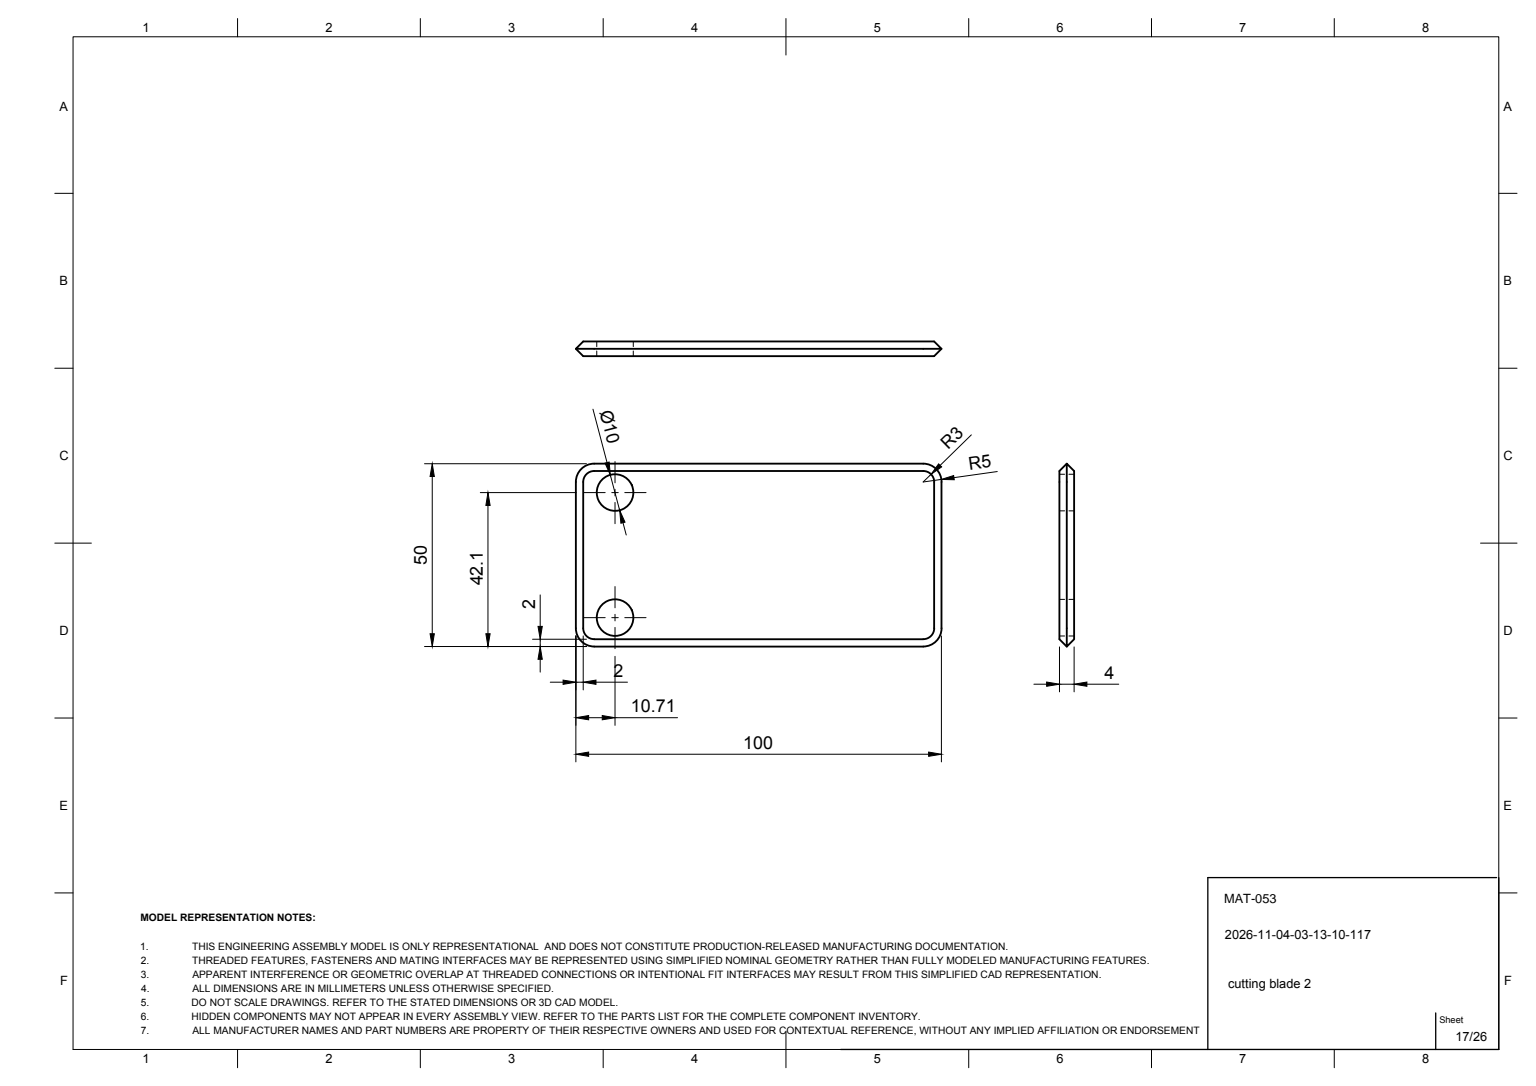
ISO-10303-21;
HEADER;
FILE_DESCRIPTION (('STEP AP214'),
    '1' );
FILE_NAME ('cutting blade 2.step',
    '2026-10-10T03:43:58',
    ( '' ),
    ( '' ),
    'SwSTEP 2.0',
    'SolidWorks 2026',
    '' );
FILE_SCHEMA (( 'AUTOMOTIVE_DESIGN' ));
ENDSEC;

DATA;
#183=ORIENTED_EDGE ( 'NONE', *, *, #3422, .F. ) ;
#222=LINE ( 'NONE', #22031, #68846 ) ;
#377=FACE_OUTER_BOUND ( 'NONE', #67584, .T. ) ;
#390=DIRECTION ( 'NONE',  ( 1.000000000000000000, 0.000000000000000000, 0.000000000000000000 ) ) ;
#471=LINE ( 'NONE', #21919, #18113 ) ;
#708=CARTESIAN_POINT ( 'NONE',  ( -48.00000000000000000, 19.99999999999996447, 0.000000000000000000 ) ) ;
#750=CARTESIAN_POINT ( 'NONE',  ( 44.99999999999997158, 22.99999999999998579, 0.000000000000000000 ) ) ;
#923=DIRECTION ( 'NONE',  ( -0.7071067811865463515, 0.000000000000000000, -0.7071067811865487940 ) ) ;
#986=EDGE_CURVE ( 'NONE', #12560, #40674, #59640, .T. ) ;
#1018=ORIENTED_EDGE ( 'NONE', *, *, #5991, .T. ) ;
#1098=DIRECTION ( 'NONE',  ( -4.906538933386759377E-15, 0.7071067811865474617, 0.7071067811865474617 ) ) ;
#1150=EDGE_LOOP ( 'NONE', ( #20877, #65074, #12430, #64337 ) ) ;
#1202=DIRECTION ( 'NONE',  ( 0.000000000000000000, 1.000000000000000000, -0.000000000000000000 ) ) ;
#1336=DIRECTION ( 'NONE',  ( 1.000000000000000000, 0.000000000000000000, 0.000000000000000000 ) ) ;
#1358=CARTESIAN_POINT ( 'NONE',  ( 49.99999999999998579, -19.99999999999996447, 2.000000000000015543 ) ) ;
#1404=DIRECTION ( 'NONE',  ( -0.000000000000000000, -0.000000000000000000, 1.000000000000000000 ) ) ;
#1589=CIRCLE ( 'NONE', #19567, 4.999999999999997335 ) ;
#1634=VECTOR ( 'NONE', #40606, 1000.000000000000114 ) ;
#1690=ORIENTED_EDGE ( 'NONE', *, *, #44656, .F. ) ;
#1791=AXIS2_PLACEMENT_3D ( 'NONE', #65034, #34080, #59734 ) ;
#2120=VERTEX_POINT ( 'NONE', #13833 ) ;
#2139=CARTESIAN_POINT ( 'NONE',  ( -44.29440389294402536, -17.09499999999999886, 0.000000000000000000 ) ) ;
#2256=EDGE_LOOP ( 'NONE', ( #42855, #11599, #67261, #3883 ) ) ;
#2297=CARTESIAN_POINT ( 'NONE',  ( 44.99999999999995737, -25.00000000000000000, 1.999999999999984457 ) ) ;
#2427=ORIENTED_EDGE ( 'NONE', *, *, #48014, .T. ) ;
#2635=CARTESIAN_POINT ( 'NONE',  ( -34.29440389294403246, 17.09499999999999886, 0.000000000000000000 ) ) ;
#2643=AXIS2_PLACEMENT_3D ( 'NONE', #60950, #23670, #66257 ) ;
#2797=CARTESIAN_POINT ( 'NONE',  ( -50.00000000000001421, -20.00000000000000355, 2.000000000000015543 ) ) ;
#2853=DIRECTION ( 'NONE',  ( -0.000000000000000000, -0.000000000000000000, -1.000000000000000000 ) ) ;
#2867=EDGE_LOOP ( 'NONE', ( #46115, #49842, #4255, #13345, #54855, #50718, #48598, #4064 ) ) ;
#2964=DIRECTION ( 'NONE',  ( -0.000000000000000000, -0.000000000000000000, -1.000000000000000000 ) ) ;
#3009=CARTESIAN_POINT ( 'NONE',  ( 44.99999999999995737, 25.00000000000000000, 1.999999999999984457 ) ) ;
#3125=CARTESIAN_POINT ( 'NONE',  ( 44.99999999999999289, -20.00000000000000355, 0.000000000000000000 ) ) ;
#3311=AXIS2_PLACEMENT_3D ( 'NONE', #56545, #46328, #29819 ) ;
#3422=EDGE_CURVE ( 'NONE', #60851, #22871, #1589, .T. ) ;
#3529=DIRECTION ( 'NONE',  ( -0.7071067811865474617, -4.906538933386759377E-15, 0.7071067811865474617 ) ) ;
#3745=AXIS2_PLACEMENT_3D ( 'NONE', #53453, #68615, #21797 ) ;
#3883=ORIENTED_EDGE ( 'NONE', *, *, #65380, .F. ) ;
#4036=EDGE_CURVE ( 'NONE', #50267, #15307, #38531, .T. ) ;
#4064=ORIENTED_EDGE ( 'NONE', *, *, #62499, .T. ) ;
#4223=CIRCLE ( 'NONE', #47977, 4.999999999999997335 ) ;
#4244=VERTEX_POINT ( 'NONE', #15155 ) ;
#4255=ORIENTED_EDGE ( 'NONE', *, *, #21903, .T. ) ;
#4322=ADVANCED_FACE ( 'NONE', ( #27075 ), #64387, .T. ) ;
#4732=CIRCLE ( 'NONE', #44038, 4.999999999999997335 ) ;
#4762=ORIENTED_EDGE ( 'NONE', *, *, #33113, .F. ) ;
#4799=VECTOR ( 'NONE', #923, 1000.000000000000000 ) ;
#4847=ADVANCED_FACE ( 'NONE', ( #5297 ), #68957, .T. ) ;
#4868=ADVANCED_FACE ( 'NONE', ( #22170 ), #20779, .T. ) ;
#4880=CARTESIAN_POINT ( 'NONE',  ( -39.29440389294403246, -17.09499999999999886, 4.000000000000000000 ) ) ;
#4934=CARTESIAN_POINT ( 'NONE',  ( -44.99999999999998579, 25.00000000000000000, 1.999999999999984457 ) ) ;
#4944=VERTEX_POINT ( 'NONE', #59784 ) ;
#5118=VECTOR ( 'NONE', #13219, 1000.000000000000114 ) ;
#5158=EDGE_CURVE ( 'NONE', #15307, #27145, #61873, .T. ) ;
#5229=DIRECTION ( 'NONE',  ( 0.000000000000000000, 0.000000000000000000, 1.000000000000000000 ) ) ;
#5297=FACE_OUTER_BOUND ( 'NONE', #5578, .T. ) ;
#5578=EDGE_LOOP ( 'NONE', ( #1690, #69065, #8868, #53921 ) ) ;
#5608=CARTESIAN_POINT ( 'NONE',  ( -45.00000000000002132, -20.00000000000000355, 2.000000000000015543 ) ) ;
#5732=CIRCLE ( 'NONE', #61882, 4.999999999999997335 ) ;
#5991=EDGE_CURVE ( 'NONE', #38832, #12486, #8955, .T. ) ;
#6249=EDGE_LOOP ( 'NONE', ( #30382, #9819, #17773, #59788 ) ) ;
#6275=DIRECTION ( 'NONE',  ( 0.000000000000000000, -1.000000000000000000, 0.000000000000000000 ) ) ;
#6382=CARTESIAN_POINT ( 'NONE',  ( -50.00000000000001421, 19.99999999999996447, 1.999999999999984457 ) ) ;
#6523=DIRECTION ( 'NONE',  ( -1.000000000000000000, 0.000000000000000000, 0.000000000000000000 ) ) ;
#6705=DIRECTION ( 'NONE',  ( -0.000000000000000000, -0.000000000000000000, -1.000000000000000000 ) ) ;
#6931=PRODUCT_CONTEXT ( 'NONE', #28708, 'mechanical' ) ;
#6943=DIRECTION ( 'NONE',  ( -1.000000000000000000, 0.000000000000000000, 0.000000000000000000 ) ) ;
#7122=CARTESIAN_POINT ( 'NONE',  ( 44.99999999999995737, -25.00000000000000000, 1.999999999999984457 ) ) ;
#7235=EDGE_CURVE ( 'NONE', #28864, #10266, #16985, .T. ) ;
#7533=DIRECTION ( 'NONE',  ( -0.000000000000000000, 0.7071067811865475727, 0.7071067811865475727 ) ) ;
#7537=VERTEX_POINT ( 'NONE', #53319 ) ;
#7773=DIRECTION ( 'NONE',  ( -0.000000000000000000, -0.000000000000000000, 1.000000000000000000 ) ) ;
#7845=CARTESIAN_POINT ( 'NONE',  ( -45.00000000000002132, 20.00000000000000355, 2.000000000000015543 ) ) ;
#7877=LINE ( 'NONE', #61339, #37506 ) ;
#7900=DIRECTION ( 'NONE',  ( 1.000000000000000000, 0.000000000000000000, 0.000000000000000000 ) ) ;
#8025=CARTESIAN_POINT ( 'NONE',  ( -34.29440389294403246, 17.09499999999999886, 4.000000000000000000 ) ) ;
#8072=CARTESIAN_POINT ( 'NONE',  ( -34.29440389294403246, -17.09499999999999886, 4.000000000000000000 ) ) ;
#8319=DIRECTION ( 'NONE',  ( 1.000000000000000000, 0.000000000000000000, 0.000000000000000000 ) ) ;
#8398=FACE_BOUND ( 'NONE', #48504, .T. ) ;
#8425=EDGE_CURVE ( 'NONE', #35305, #28864, #65814, .T. ) ;
#8459=AXIS2_PLACEMENT_3D ( 'NONE', #30320, #9554, #52459 ) ;
#8475=SURFACE_STYLE_FILL_AREA ( #51035 ) ;
#8515=VECTOR ( 'NONE', #8859, 1000.000000000000114 ) ;
#8610=CYLINDRICAL_SURFACE ( 'NONE', #31391, 4.999999999999997335 ) ;
#8770=( NAMED_UNIT ( * ) SI_UNIT ( $, .STERADIAN. ) SOLID_ANGLE_UNIT ( ) );
#8823=ORIENTED_EDGE ( 'NONE', *, *, #5158, .T. ) ;
#8843=CARTESIAN_POINT ( 'NONE',  ( -34.29440389294403246, -17.09499999999999886, 4.000000000000000000 ) ) ;
#8859=DIRECTION ( 'NONE',  ( 0.7071067811865474617, 0.000000000000000000, -0.7071067811865474617 ) ) ;
#8868=ORIENTED_EDGE ( 'NONE', *, *, #31433, .F. ) ;
#8955=LINE ( 'NONE', #2297, #1634 ) ;
#9255=ORIENTED_EDGE ( 'NONE', *, *, #36424, .T. ) ;
#9426=AXIS2_PLACEMENT_3D ( 'NONE', #64039, #26413, #64375 ) ;
#9467=CONICAL_SURFACE ( 'NONE', #13979, 4.999999999999997335, 0.7853981633974482790 ) ;
#9554=DIRECTION ( 'NONE',  ( 0.000000000000000000, 0.000000000000000000, -1.000000000000000000 ) ) ;
#9615=VECTOR ( 'NONE', #7900, 1000.000000000000000 ) ;
#9738=LINE ( 'NONE', #67202, #34763 ) ;
#9744=ORIENTED_EDGE ( 'NONE', *, *, #46447, .T. ) ;
#9800=ORIENTED_EDGE ( 'NONE', *, *, #50666, .T. ) ;
#9819=ORIENTED_EDGE ( 'NONE', *, *, #48014, .F. ) ;
#10092=CARTESIAN_POINT ( 'NONE',  ( 47.99999999999997158, 19.99999999999996447, 4.000000000000000000 ) ) ;
#10095=CIRCLE ( 'NONE', #43771, 4.999999999999997335 ) ;
#10266=VERTEX_POINT ( 'NONE', #11721 ) ;
#10705=PLANE ( 'NONE',  #20640 ) ;
#11124=DIRECTION ( 'NONE',  ( -0.7071067811865474617, 0.000000000000000000, 0.7071067811865474617 ) ) ;
#11164=CARTESIAN_POINT ( 'NONE',  ( 47.99999999999997158, 19.99999999999996447, 4.000000000000000000 ) ) ;
#11274=CARTESIAN_POINT ( 'NONE',  ( -34.29440389294403246, 17.09499999999999886, 4.000000000000000000 ) ) ;
#11390=CARTESIAN_POINT ( 'NONE',  ( 49.99999999999998579, -19.99999999999996447, 2.000000000000015543 ) ) ;
#11409=DIRECTION ( 'NONE',  ( 0.000000000000000000, 1.000000000000000000, 0.000000000000000000 ) ) ;
#11454=CARTESIAN_POINT ( 'NONE',  ( -48.00000000000000711, -20.00000000000000355, 4.000000000000000000 ) ) ;
#11599=ORIENTED_EDGE ( 'NONE', *, *, #4036, .F. ) ;
#11721=CARTESIAN_POINT ( 'NONE',  ( -44.29440389294402536, 17.09499999999999886, 0.000000000000000000 ) ) ;
#11786=FACE_OUTER_BOUND ( 'NONE', #1150, .T. ) ;
#11882=DIRECTION ( 'NONE',  ( 0.000000000000000000, 0.000000000000000000, 1.000000000000000000 ) ) ;
#12224=CARTESIAN_POINT ( 'NONE',  ( 44.99999999999999289, 20.00000000000000355, 4.000000000000000000 ) ) ;
#12325=VECTOR ( 'NONE', #37666, 1000.000000000000000 ) ;
#12430=ORIENTED_EDGE ( 'NONE', *, *, #5991, .F. ) ;
#12479=DIRECTION ( 'NONE',  ( 4.906538933386759377E-15, 0.7071067811865474617, -0.7071067811865474617 ) ) ;
#12486=VERTEX_POINT ( 'NONE', #28146 ) ;
#12522=VECTOR ( 'NONE', #11409, 1000.000000000000000 ) ;
#12560=VERTEX_POINT ( 'NONE', #44325 ) ;
#12589=ORIENTED_EDGE ( 'NONE', *, *, #62499, .F. ) ;
#12741=DIRECTION ( 'NONE',  ( 0.000000000000000000, 0.000000000000000000, 1.000000000000000000 ) ) ;
#12788=EDGE_CURVE ( 'NONE', #35305, #62075, #59114, .T. ) ;
#12803=CARTESIAN_POINT ( 'NONE',  ( -44.99999999999998579, -25.00000000000000000, 2.000000000000015543 ) ) ;
#12850=DIRECTION ( 'NONE',  ( -0.000000000000000000, -0.000000000000000000, -1.000000000000000000 ) ) ;
#12851=VERTEX_POINT ( 'NONE', #22536 ) ;
#12994=CARTESIAN_POINT ( 'NONE',  ( -44.99999999999998579, 25.00000000000000000, 2.000000000000015543 ) ) ;
#13009=ORIENTED_EDGE ( 'NONE', *, *, #49203, .T. ) ;
#13019=FACE_OUTER_BOUND ( 'NONE', #6249, .T. ) ;
#13037=DIRECTION ( 'NONE',  ( -0.000000000000000000, -0.000000000000000000, 1.000000000000000000 ) ) ;
#13138=FACE_OUTER_BOUND ( 'NONE', #28425, .T. ) ;
#13214=EDGE_CURVE ( 'NONE', #16065, #15985, #21273, .T. ) ;
#13219=DIRECTION ( 'NONE',  ( 4.906538933386759377E-15, -0.7071067811865474617, 0.7071067811865474617 ) ) ;
#13345=ORIENTED_EDGE ( 'NONE', *, *, #48539, .T. ) ;
#13488=AXIS2_PLACEMENT_3D ( 'NONE', #22899, #7773, #17980 ) ;
#13502=EDGE_CURVE ( 'NONE', #63560, #2120, #43992, .T. ) ;
#13538=CARTESIAN_POINT ( 'NONE',  ( -44.99999999999998579, 25.00000000000000000, 2.000000000000015543 ) ) ;
#13780=CARTESIAN_POINT ( 'NONE',  ( 44.99999999999999289, -20.00000000000000355, 2.000000000000015543 ) ) ;
#13831=DIRECTION ( 'NONE',  ( 0.000000000000000000, 0.000000000000000000, 1.000000000000000000 ) ) ;
#13833=CARTESIAN_POINT ( 'NONE',  ( 44.99999999999995737, 25.00000000000000000, 1.999999999999984457 ) ) ;
#13881=EDGE_CURVE ( 'NONE', #4944, #25496, #66247, .T. ) ;
#13979=AXIS2_PLACEMENT_3D ( 'NONE', #5608, #47479, #52756 ) ;
#14090=LINE ( 'NONE', #52413, #14981 ) ;
#14258=PLANE ( 'NONE',  #28801 ) ;
#14352=DIRECTION ( 'NONE',  ( 0.000000000000000000, -0.7071067811865474617, -0.7071067811865474617 ) ) ;
#14380=AXIS2_PLACEMENT_3D ( 'NONE', #24758, #63424, #57113 ) ;
#14790=AXIS2_PLACEMENT_3D ( 'NONE', #30257, #24641, #63650 ) ;
#14981=VECTOR ( 'NONE', #3529, 1000.000000000000114 ) ;
#14989=ORIENTED_EDGE ( 'NONE', *, *, #7235, .T. ) ;
#14998=ADVANCED_FACE ( 'NONE', ( #61511, #8398, #60802 ), #50261, .F. ) ;
#15004=DIRECTION ( 'NONE',  ( 0.000000000000000000, -1.000000000000000000, 0.000000000000000000 ) ) ;
#15155=CARTESIAN_POINT ( 'NONE',  ( -44.99999999999998579, -25.00000000000000000, 1.999999999999984457 ) ) ;
#15307=VERTEX_POINT ( 'NONE', #60726 ) ;
#15476=SURFACE_STYLE_USAGE ( .BOTH. , #52740 ) ;
#15509=EDGE_LOOP ( 'NONE', ( #32307, #42326, #26888, #23575 ) ) ;
#15809=PRESENTATION_STYLE_ASSIGNMENT (( #15476 ) ) ;
#15831=AXIS2_PLACEMENT_3D ( 'NONE', #19106, #13831, #18417 ) ;
#15947=CLOSED_SHELL ( 'NONE', ( #32652, #33942, #58809, #14998, #32048, #67428, #50501, #38188, #4847, #4322, #43169, #65687, #64587, #40447, #23137, #4868, #26968, #20171, #36132, #26544, #66069, #55190 ) ) ;
#15985=VERTEX_POINT ( 'NONE', #68162 ) ;
#16065=VERTEX_POINT ( 'NONE', #10092 ) ;
#16112=EDGE_LOOP ( 'NONE', ( #27726, #56434 ) ) ;
#16253=PRODUCT_DEFINITION_CONTEXT ( 'detailed design', #53830, 'design' ) ;
#16512=ORIENTED_EDGE ( 'NONE', *, *, #32179, .T. ) ;
#16541=FACE_OUTER_BOUND ( 'NONE', #31950, .T. ) ;
#16985=LINE ( 'NONE', #49686, #46669 ) ;
#17050=CARTESIAN_POINT ( 'NONE',  ( 47.99999999999997158, -19.99999999999997868, 0.000000000000000000 ) ) ;
#17127=EDGE_CURVE ( 'NONE', #25708, #50267, #25270, .T. ) ;
#17166=COLOUR_RGB ( '',0.7921568627450980005, 0.8196078431372548767, 0.9333333333333333481 ) ;
#17773=ORIENTED_EDGE ( 'NONE', *, *, #25587, .F. ) ;
#17789=VECTOR ( 'NONE', #12479, 1000.000000000000114 ) ;
#17937=DIRECTION ( 'NONE',  ( -0.000000000000000000, -0.000000000000000000, -1.000000000000000000 ) ) ;
#17980=DIRECTION ( 'NONE',  ( 1.000000000000000000, 0.000000000000000000, 0.000000000000000000 ) ) ;
#18104=CARTESIAN_POINT ( 'NONE',  ( 44.99999999999995737, -22.99999999999998579, 4.000000000000000000 ) ) ;
#18113=VECTOR ( 'NONE', #44422, 1000.000000000000114 ) ;
#18224=DIRECTION ( 'NONE',  ( 0.000000000000000000, -1.000000000000000000, 0.000000000000000000 ) ) ;
#18228=ORIENTED_EDGE ( 'NONE', *, *, #51150, .F. ) ;
#18296=FACE_OUTER_BOUND ( 'NONE', #2256, .T. ) ;
#18356=EDGE_CURVE ( 'NONE', #40674, #18627, #20345, .T. ) ;
#18417=DIRECTION ( 'NONE',  ( 1.000000000000000000, 0.000000000000000000, 0.000000000000000000 ) ) ;
#18522=DIRECTION ( 'NONE',  ( -0.000000000000000000, -0.000000000000000000, 1.000000000000000000 ) ) ;
#18580=CARTESIAN_POINT ( 'NONE',  ( -45.00000000000002132, 20.00000000000000355, 4.000000000000000000 ) ) ;
#18627=VERTEX_POINT ( 'NONE', #41386 ) ;
#18718=DIRECTION ( 'NONE',  ( 1.000000000000000000, 0.000000000000000000, 0.000000000000000000 ) ) ;
#18762=ORIENTED_EDGE ( 'NONE', *, *, #23426, .F. ) ;
#18857=ORIENTED_EDGE ( 'NONE', *, *, #13881, .F. ) ;
#18879=SHAPE_DEFINITION_REPRESENTATION ( #51752, #64096 ) ;
#19106=CARTESIAN_POINT ( 'NONE',  ( -39.29440389294403246, -17.09499999999999886, 0.000000000000000000 ) ) ;
#19194=CIRCLE ( 'NONE', #59591, 4.999999999999997335 ) ;
#19282=DIRECTION ( 'NONE',  ( 0.000000000000000000, 0.000000000000000000, 1.000000000000000000 ) ) ;
#19376=CARTESIAN_POINT ( 'NONE',  ( -44.29440389294402536, 17.09499999999999886, 4.000000000000000000 ) ) ;
#19480=CARTESIAN_POINT ( 'NONE',  ( -45.00000000000000000, 22.99999999999998579, 4.000000000000000000 ) ) ;
#19491=CARTESIAN_POINT ( 'NONE',  ( -39.29440389294403246, -17.09499999999999886, 4.000000000000000000 ) ) ;
#19560=CARTESIAN_POINT ( 'NONE',  ( -44.99999999999998579, -25.00000000000000000, 2.000000000000015543 ) ) ;
#19567=AXIS2_PLACEMENT_3D ( 'NONE', #54925, #60906, #28914 ) ;
#19604=CARTESIAN_POINT ( 'NONE',  ( -50.00000000000001421, -19.99999999999996447, 2.000000000000015543 ) ) ;
#19746=LINE ( 'NONE', #57045, #8515 ) ;
#19766=LINE ( 'NONE', #56710, #40477 ) ;
#19850=PLANE ( 'NONE',  #63041 ) ;
#19933=EDGE_LOOP ( 'NONE', ( #24188, #34340, #56345, #65370 ) ) ;
#20171=ADVANCED_FACE ( 'NONE', ( #18296 ), #55242, .T. ) ;
#20217=DIRECTION ( 'NONE',  ( 0.000000000000000000, 0.000000000000000000, 1.000000000000000000 ) ) ;
#20278=EDGE_CURVE ( 'NONE', #22871, #60851, #4732, .T. ) ;
#20345=LINE ( 'NONE', #2797, #41653 ) ;
#20428=CARTESIAN_POINT ( 'NONE',  ( 47.99999999999997158, 19.99999999999996447, 0.000000000000000000 ) ) ;
#20585=CARTESIAN_POINT ( 'NONE',  ( 47.99999999999997158, 19.99999999999996447, 0.000000000000000000 ) ) ;
#20640=AXIS2_PLACEMENT_3D ( 'NONE', #11390, #49018, #1202 ) ;
#20779=PLANE ( 'NONE',  #28501 ) ;
#20844=VECTOR ( 'NONE', #62363, 1000.000000000000114 ) ;
#20877=ORIENTED_EDGE ( 'NONE', *, *, #67680, .T. ) ;
#20898=EDGE_LOOP ( 'NONE', ( #47431, #46905, #14989, #35358 ) ) ;
#20942=VECTOR ( 'NONE', #33017, 1000.000000000000000 ) ;
#21176=VERTEX_POINT ( 'NONE', #25603 ) ;
#21178=ORIENTED_EDGE ( 'NONE', *, *, #40498, .T. ) ;
#21271=EDGE_CURVE ( 'NONE', #42749, #16065, #222, .T. ) ;
#21273=CIRCLE ( 'NONE', #3311, 2.999999999999981792 ) ;
#21355=ORIENTED_EDGE ( 'NONE', *, *, #34936, .F. ) ;
#21466=DIRECTION ( 'NONE',  ( 0.000000000000000000, 1.000000000000000000, 0.000000000000000000 ) ) ;
#21508=ORIENTED_EDGE ( 'NONE', *, *, #36424, .F. ) ;
#21797=DIRECTION ( 'NONE',  ( 1.000000000000000000, 0.000000000000000000, 0.000000000000000000 ) ) ;
#21854=ORIENTED_EDGE ( 'NONE', *, *, #13502, .F. ) ;
#21903=EDGE_CURVE ( 'NONE', #12486, #21176, #62173, .T. ) ;
#21919=CARTESIAN_POINT ( 'NONE',  ( -44.99999999999998579, 25.00000000000000000, 2.000000000000015543 ) ) ;
#21973=LINE ( 'NONE', #65961, #12522 ) ;
#22005=AXIS2_PLACEMENT_3D ( 'NONE', #32747, #34156, #27111 ) ;
#22031=CARTESIAN_POINT ( 'NONE',  ( 49.99999999999998579, 19.99999999999996447, 1.999999999999984457 ) ) ;
#22079=DIRECTION ( 'NONE',  ( -0.000000000000000000, -0.000000000000000000, -1.000000000000000000 ) ) ;
#22170=FACE_OUTER_BOUND ( 'NONE', #63972, .T. ) ;
#22536=CARTESIAN_POINT ( 'NONE',  ( -45.00000000000000000, 22.99999999999998579, 0.000000000000000000 ) ) ;
#22658=UNCERTAINTY_MEASURE_WITH_UNIT (LENGTH_MEASURE( 1.000000000000000082E-05 ), #50619, 'distance_accuracy_value', 'NONE');
#22858=DIRECTION ( 'NONE',  ( 1.000000000000000000, 0.000000000000000000, 0.000000000000000000 ) ) ;
#22871=VERTEX_POINT ( 'NONE', #8843 ) ;
#22899=CARTESIAN_POINT ( 'NONE',  ( -45.00000000000002132, -20.00000000000000355, 2.000000000000015543 ) ) ;
#23124=VECTOR ( 'NONE', #51323, 1000.000000000000114 ) ;
#23130=DIRECTION ( 'NONE',  ( -0.000000000000000000, -0.000000000000000000, -1.000000000000000000 ) ) ;
#23137=ADVANCED_FACE ( 'NONE', ( #13138 ), #9467, .T. ) ;
#23379=EDGE_CURVE ( 'NONE', #25708, #42749, #68770, .T. ) ;
#23426=EDGE_CURVE ( 'NONE', #4244, #38832, #45946, .T. ) ;
#23485=CYLINDRICAL_SURFACE ( 'NONE', #45903, 4.999999999999997335 ) ;
#23575=ORIENTED_EDGE ( 'NONE', *, *, #27011, .F. ) ;
#23602=FACE_OUTER_BOUND ( 'NONE', #50503, .T. ) ;
#23670=DIRECTION ( 'NONE',  ( -0.000000000000000000, -0.000000000000000000, -1.000000000000000000 ) ) ;
#23733=ORIENTED_EDGE ( 'NONE', *, *, #20278, .T. ) ;
#23738=VECTOR ( 'NONE', #31568, 1000.000000000000000 ) ;
#23823=FACE_OUTER_BOUND ( 'NONE', #62051, .T. ) ;
#23895=SHAPE_REPRESENTATION_RELATIONSHIP ( 'NONE' , 'NONE' ,  #64096, #40723 ) ;
#24022=DIRECTION ( 'NONE',  ( 1.000000000000000000, 0.000000000000000000, 0.000000000000000000 ) ) ;
#24188=ORIENTED_EDGE ( 'NONE', *, *, #3422, .T. ) ;
#24480=ORIENTED_EDGE ( 'NONE', *, *, #48539, .F. ) ;
#24585=DIRECTION ( 'NONE',  ( 1.000000000000000000, 0.000000000000000000, -0.000000000000000000 ) ) ;
#24641=DIRECTION ( 'NONE',  ( -0.000000000000000000, -0.000000000000000000, -1.000000000000000000 ) ) ;
#24758=CARTESIAN_POINT ( 'NONE',  ( -45.00000000000002132, 20.00000000000000355, 0.000000000000000000 ) ) ;
#25032=EDGE_CURVE ( 'NONE', #65565, #12486, #60661, .T. ) ;
#25166=DIRECTION ( 'NONE',  ( 0.000000000000000000, 0.000000000000000000, 1.000000000000000000 ) ) ;
#25270=LINE ( 'NONE', #30198, #23738 ) ;
#25396=DIRECTION ( 'NONE',  ( 0.000000000000000000, 0.000000000000000000, -1.000000000000000000 ) ) ;
#25496=VERTEX_POINT ( 'NONE', #65880 ) ;
#25587=EDGE_CURVE ( 'NONE', #39558, #31561, #19746, .T. ) ;
#25603=CARTESIAN_POINT ( 'NONE',  ( 47.99999999999997158, -19.99999999999997868, 4.000000000000000000 ) ) ;
#25633=CIRCLE ( 'NONE', #14380, 2.999999999999981792 ) ;
#25708=VERTEX_POINT ( 'NONE', #20428 ) ;
#25725=CIRCLE ( 'NONE', #58246, 2.999999999999981792 ) ;
#26176=MECHANICAL_DESIGN_GEOMETRIC_PRESENTATION_REPRESENTATION('',(#58740),#28427);
#26257=CARTESIAN_POINT ( 'NONE',  ( -48.00000000000000711, -20.00000000000000355, 4.000000000000000000 ) ) ;
#26413=DIRECTION ( 'NONE',  ( 0.000000000000000000, 0.7071067811865475727, 0.7071067811865475727 ) ) ;
#26495=ORIENTED_EDGE ( 'NONE', *, *, #4036, .T. ) ;
#26544=ADVANCED_FACE ( 'NONE', ( #62322 ), #50018, .T. ) ;
#26865=AXIS2_PLACEMENT_3D ( 'NONE', #12224, #49484, #66749 ) ;
#26888=ORIENTED_EDGE ( 'NONE', *, *, #18356, .F. ) ;
#26968=ADVANCED_FACE ( 'NONE', ( #23602 ), #40806, .T. ) ;
#27011=EDGE_CURVE ( 'NONE', #39558, #40674, #54448, .T. ) ;
#27075=FACE_OUTER_BOUND ( 'NONE', #67313, .T. ) ;
#27085=DIRECTION ( 'NONE',  ( 0.000000000000000000, -0.7071067811865475727, 0.7071067811865475727 ) ) ;
#27111=DIRECTION ( 'NONE',  ( 1.000000000000000000, 0.000000000000000000, 0.000000000000000000 ) ) ;
#27145=VERTEX_POINT ( 'NONE', #62091 ) ;
#27228=FACE_OUTER_BOUND ( 'NONE', #54661, .T. ) ;
#27273=AXIS2_PLACEMENT_3D ( 'NONE', #30730, #2964, #46902 ) ;
#27455=EDGE_CURVE ( 'NONE', #25496, #39558, #40907, .T. ) ;
#27726=ORIENTED_EDGE ( 'NONE', *, *, #34770, .F. ) ;
#28146=CARTESIAN_POINT ( 'NONE',  ( 44.99999999999995737, -22.99999999999998579, 4.000000000000000000 ) ) ;
#28425=EDGE_LOOP ( 'NONE', ( #35121, #67993, #48370, #21355 ) ) ;
#28427=( GEOMETRIC_REPRESENTATION_CONTEXT ( 3 ) GLOBAL_UNCERTAINTY_ASSIGNED_CONTEXT ( ( #33920 ) ) GLOBAL_UNIT_ASSIGNED_CONTEXT ( ( #53424, #30620, #41516 ) ) REPRESENTATION_CONTEXT ( 'NONE', 'WORKASPACE' ) );
#28433=LINE ( 'NONE', #1358, #20942 ) ;
#28501=AXIS2_PLACEMENT_3D ( 'NONE', #36626, #42242, #21466 ) ;
#28708=APPLICATION_CONTEXT ( 'automotive_design' ) ;
#28801=AXIS2_PLACEMENT_3D ( 'NONE', #35717, #25166, #46595 ) ;
#28844=LINE ( 'NONE', #8072, #51936 ) ;
#28864=VERTEX_POINT ( 'NONE', #19376 ) ;
#28914=DIRECTION ( 'NONE',  ( 1.000000000000000000, 0.000000000000000000, 0.000000000000000000 ) ) ;
#28943=ORIENTED_EDGE ( 'NONE', *, *, #5158, .F. ) ;
#29154=AXIS2_PLACEMENT_3D ( 'NONE', #32742, #59461, #42932 ) ;
#29202=DIRECTION ( 'NONE',  ( 0.7071067811865474617, 4.906538933386759377E-15, 0.7071067811865474617 ) ) ;
#29271=ORIENTED_EDGE ( 'NONE', *, *, #45883, .F. ) ;
#29421=ORIENTED_EDGE ( 'NONE', *, *, #67680, .F. ) ;
#29435=ORIENTED_EDGE ( 'NONE', *, *, #45883, .T. ) ;
#29570=FILL_AREA_STYLE_COLOUR ( '', #17166 ) ;
#29663=DIRECTION ( 'NONE',  ( 1.000000000000000000, 0.000000000000000000, 0.000000000000000000 ) ) ;
#29819=DIRECTION ( 'NONE',  ( 1.000000000000000000, 0.000000000000000000, 0.000000000000000000 ) ) ;
#30184=CARTESIAN_POINT ( 'NONE',  ( -44.99999999999998579, -22.99999999999998579, 4.000000000000000000 ) ) ;
#30193=ORIENTED_EDGE ( 'NONE', *, *, #43361, .F. ) ;
#30198=CARTESIAN_POINT ( 'NONE',  ( 47.99999999999997158, -20.00000000000000355, 0.000000000000000000 ) ) ;
#30257=CARTESIAN_POINT ( 'NONE',  ( 44.99999999999999289, 20.00000000000000355, 0.000000000000000000 ) ) ;
#30320=CARTESIAN_POINT ( 'NONE',  ( -45.00000000000002132, -20.00000000000000355, 4.000000000000000000 ) ) ;
#30382=ORIENTED_EDGE ( 'NONE', *, *, #51150, .T. ) ;
#30388=CONICAL_SURFACE ( 'NONE', #47191, 2.999999999999981792, 0.7853981633974482790 ) ;
#30620=( NAMED_UNIT ( * ) PLANE_ANGLE_UNIT ( ) SI_UNIT ( $, .RADIAN. ) );
#30671=DIRECTION ( 'NONE',  ( 1.000000000000000000, 0.000000000000000000, 0.000000000000000000 ) ) ;
#30708=AXIS2_PLACEMENT_3D ( 'NONE', #40558, #69275, #29663 ) ;
#30730=CARTESIAN_POINT ( 'NONE',  ( 44.99999999999999289, -20.00000000000000355, 0.000000000000000000 ) ) ;
#30780=FACE_OUTER_BOUND ( 'NONE', #2867, .T. ) ;
#31012=DIRECTION ( 'NONE',  ( -1.000000000000000000, 0.000000000000000000, 0.000000000000000000 ) ) ;
#31181=ORIENTED_EDGE ( 'NONE', *, *, #23426, .T. ) ;
#31391=AXIS2_PLACEMENT_3D ( 'NONE', #19491, #12850, #55749 ) ;
#31432=ORIENTED_EDGE ( 'NONE', *, *, #7235, .F. ) ;
#31433=EDGE_CURVE ( 'NONE', #4944, #48269, #51510, .T. ) ;
#31561=VERTEX_POINT ( 'NONE', #708 ) ;
#31568=DIRECTION ( 'NONE',  ( 0.000000000000000000, -1.000000000000000000, 0.000000000000000000 ) ) ;
#31687=CARTESIAN_POINT ( 'NONE',  ( -45.00000000000002132, 20.00000000000000355, 4.000000000000000000 ) ) ;
#31937=EDGE_LOOP ( 'NONE', ( #28943, #59280, #18762, #21178 ) ) ;
#31950=EDGE_LOOP ( 'NONE', ( #63608, #31181, #1018, #43485 ) ) ;
#32009=ORIENTED_EDGE ( 'NONE', *, *, #58117, .T. ) ;
#32048=ADVANCED_FACE ( 'NONE', ( #54413 ), #23485, .F. ) ;
#32066=DIRECTION ( 'NONE',  ( 0.000000000000000000, 0.000000000000000000, 1.000000000000000000 ) ) ;
#32179=EDGE_CURVE ( 'NONE', #27145, #18627, #25725, .T. ) ;
#32207=ORIENTED_EDGE ( 'NONE', *, *, #12788, .T. ) ;
#32238=VECTOR ( 'NONE', #2853, 1000.000000000000000 ) ;
#32307=ORIENTED_EDGE ( 'NONE', *, *, #25587, .T. ) ;
#32652=ADVANCED_FACE ( 'NONE', ( #61023 ), #8610, .F. ) ;
#32723=PLANE ( 'NONE',  #55498 ) ;
#32742=CARTESIAN_POINT ( 'NONE',  ( -39.29440389294403246, 17.09499999999999886, 4.000000000000000000 ) ) ;
#32747=CARTESIAN_POINT ( 'NONE',  ( -45.00000000000002132, -20.00000000000000355, 4.000000000000000000 ) ) ;
#33015=CARTESIAN_POINT ( 'NONE',  ( -50.00000000000001421, -19.99999999999996447, 2.000000000000015543 ) ) ;
#33017=DIRECTION ( 'NONE',  ( 0.000000000000000000, 1.000000000000000000, 0.000000000000000000 ) ) ;
#33062=VECTOR ( 'NONE', #41019, 1000.000000000000000 ) ;
#33077=ORIENTED_EDGE ( 'NONE', *, *, #52632, .F. ) ;
#33113=EDGE_CURVE ( 'NONE', #50267, #7537, #9738, .T. ) ;
#33262=DIRECTION ( 'NONE',  ( 0.000000000000000000, 0.000000000000000000, -1.000000000000000000 ) ) ;
#33703=EDGE_LOOP ( 'NONE', ( #21854, #52340, #18228, #65805 ) ) ;
#33920=UNCERTAINTY_MEASURE_WITH_UNIT (LENGTH_MEASURE( 1.000000000000000082E-05 ), #53424, 'distance_accuracy_value', 'NONE');
#33942=ADVANCED_FACE ( 'NONE', ( #377 ), #43279, .F. ) ;
#34056=EDGE_CURVE ( 'NONE', #15985, #4944, #64399, .T. ) ;
#34064=VERTEX_POINT ( 'NONE', #2139 ) ;
#34080=DIRECTION ( 'NONE',  ( 0.000000000000000000, 0.000000000000000000, 1.000000000000000000 ) ) ;
#34156=DIRECTION ( 'NONE',  ( 0.000000000000000000, 0.000000000000000000, 1.000000000000000000 ) ) ;
#34170=ORIENTED_EDGE ( 'NONE', *, *, #20278, .F. ) ;
#34259=FACE_OUTER_BOUND ( 'NONE', #31937, .T. ) ;
#34340=ORIENTED_EDGE ( 'NONE', *, *, #38178, .T. ) ;
#34365=DIRECTION ( 'NONE',  ( 1.000000000000000000, 0.000000000000000000, 0.000000000000000000 ) ) ;
#34389=CIRCLE ( 'NONE', #22005, 2.999999999999981792 ) ;
#34500=DIRECTION ( 'NONE',  ( 1.000000000000000000, 0.000000000000000000, 0.000000000000000000 ) ) ;
#34763=VECTOR ( 'NONE', #29202, 1000.000000000000114 ) ;
#34770=EDGE_CURVE ( 'NONE', #28864, #35305, #55043, .T. ) ;
#34854=DIRECTION ( 'NONE',  ( 0.7071067811865475727, 0.000000000000000000, 0.7071067811865475727 ) ) ;
#34936=EDGE_CURVE ( 'NONE', #40674, #4244, #62897, .T. ) ;
#34951=PLANE ( 'NONE',  #55138 ) ;
#34993=DIRECTION ( 'NONE',  ( -1.000000000000000000, 0.000000000000000000, 0.000000000000000000 ) ) ;
#35121=ORIENTED_EDGE ( 'NONE', *, *, #18356, .T. ) ;
#35135=ORIENTED_EDGE ( 'NONE', *, *, #34770, .T. ) ;
#35305=VERTEX_POINT ( 'NONE', #8025 ) ;
#35358=ORIENTED_EDGE ( 'NONE', *, *, #50666, .F. ) ;
#35406=ORIENTED_EDGE ( 'NONE', *, *, #58413, .F. ) ;
#35517=ORIENTED_EDGE ( 'NONE', *, *, #51624, .T. ) ;
#35540=DIRECTION ( 'NONE',  ( 0.000000000000000000, -1.000000000000000000, 0.000000000000000000 ) ) ;
#35619=ORIENTED_EDGE ( 'NONE', *, *, #27011, .T. ) ;
#35717=CARTESIAN_POINT ( 'NONE',  ( 44.99999999999999289, -20.00000000000000355, 4.000000000000000000 ) ) ;
#35731=EDGE_LOOP ( 'NONE', ( #26495, #8823, #16512, #58515, #2427, #36975, #35517, #55410 ) ) ;
#36027=CIRCLE ( 'NONE', #15831, 4.999999999999997335 ) ;
#36079=EDGE_CURVE ( 'NONE', #34064, #51605, #36027, .T. ) ;
#36132=ADVANCED_FACE ( 'NONE', ( #34259 ), #34951, .F. ) ;
#36221=CARTESIAN_POINT ( 'NONE',  ( -34.29440389294403246, -17.09499999999999886, 0.000000000000000000 ) ) ;
#36402=ORIENTED_EDGE ( 'NONE', *, *, #23379, .T. ) ;
#36424=EDGE_CURVE ( 'NONE', #42749, #2120, #19194, .T. ) ;
#36536=DIRECTION ( 'NONE',  ( 0.7071067811865463515, 0.000000000000000000, -0.7071067811865487940 ) ) ;
#36626=CARTESIAN_POINT ( 'NONE',  ( -48.00000000000000711, -20.00000000000000355, 4.000000000000000000 ) ) ;
#36975=ORIENTED_EDGE ( 'NONE', *, *, #66483, .T. ) ;
#37074=AXIS2_PLACEMENT_3D ( 'NONE', #64767, #32066, #390 ) ;
#37236=EDGE_CURVE ( 'NONE', #18627, #31561, #21973, .T. ) ;
#37506=VECTOR ( 'NONE', #55354, 1000.000000000000114 ) ;
#37599=AXIS2_PLACEMENT_3D ( 'NONE', #19604, #55865, #18224 ) ;
#37629=ORIENTED_EDGE ( 'NONE', *, *, #51624, .F. ) ;
#37642=DIRECTION ( 'NONE',  ( -1.000000000000000000, 0.000000000000000000, 0.000000000000000000 ) ) ;
#37666=DIRECTION ( 'NONE',  ( -1.000000000000000000, 0.000000000000000000, 0.000000000000000000 ) ) ;
#38178=EDGE_CURVE ( 'NONE', #22871, #51605, #28844, .T. ) ;
#38188=ADVANCED_FACE ( 'NONE', ( #13019 ), #50780, .T. ) ;
#38348=ORIENTED_EDGE ( 'NONE', *, *, #27455, .T. ) ;
#38455=DIRECTION ( 'NONE',  ( -0.000000000000000000, -0.000000000000000000, -1.000000000000000000 ) ) ;
#38531=CIRCLE ( 'NONE', #27273, 2.999999999999981792 ) ;
#38612=CARTESIAN_POINT ( 'NONE',  ( -44.99999999999998579, -22.99999999999998579, 4.000000000000000000 ) ) ;
#38810=FACE_OUTER_BOUND ( 'NONE', #46314, .T. ) ;
#38832=VERTEX_POINT ( 'NONE', #7122 ) ;
#39124=ORIENTED_EDGE ( 'NONE', *, *, #21271, .T. ) ;
#39135=CARTESIAN_POINT ( 'NONE',  ( -39.29440389294403246, 17.09499999999999886, 0.000000000000000000 ) ) ;
#39324=CARTESIAN_POINT ( 'NONE',  ( -39.29440389294403246, 17.09499999999999886, 0.000000000000000000 ) ) ;
#39558=VERTEX_POINT ( 'NONE', #6382 ) ;
#39737=CARTESIAN_POINT ( 'NONE',  ( -45.00000000000002132, 20.00000000000000355, 2.000000000000015543 ) ) ;
#39756=CARTESIAN_POINT ( 'NONE',  ( 44.99999999999999289, -20.00000000000000355, 2.000000000000015543 ) ) ;
#39790=MANIFOLD_SOLID_BREP ( 'Chamfer1', #15947 ) ;
#40071=( NAMED_UNIT ( * ) PLANE_ANGLE_UNIT ( ) SI_UNIT ( $, .RADIAN. ) );
#40447=ADVANCED_FACE ( 'NONE', ( #27228 ), #10705, .F. ) ;
#40477=VECTOR ( 'NONE', #30671, 1000.000000000000000 ) ;
#40498=EDGE_CURVE ( 'NONE', #4244, #27145, #7877, .T. ) ;
#40558=CARTESIAN_POINT ( 'NONE',  ( 44.99999999999999289, -20.00000000000000355, 4.000000000000000000 ) ) ;
#40606=DIRECTION ( 'NONE',  ( 0.000000000000000000, 0.7071067811865474617, 0.7071067811865474617 ) ) ;
#40674=VERTEX_POINT ( 'NONE', #62019 ) ;
#40706=PLANE ( 'NONE',  #37599 ) ;
#40723=ADVANCED_BREP_SHAPE_REPRESENTATION ( '', ( #39790, #66832 ), #44451 ) ;
#40806=PLANE ( 'NONE',  #57858 ) ;
#40907=LINE ( 'NONE', #68001, #20844 ) ;
#40956=FACE_OUTER_BOUND ( 'NONE', #33703, .T. ) ;
#40981=FACE_BOUND ( 'NONE', #16112, .T. ) ;
#41019=DIRECTION ( 'NONE',  ( 1.000000000000000000, 0.000000000000000000, 0.000000000000000000 ) ) ;
#41145=PRODUCT_DEFINITION_FORMATION_WITH_SPECIFIED_SOURCE ( 'ANY', '', #59083, .NOT_KNOWN. ) ;
#41386=CARTESIAN_POINT ( 'NONE',  ( -48.00000000000000711, -20.00000000000000355, 0.000000000000000000 ) ) ;
#41502=EDGE_LOOP ( 'NONE', ( #51708, #32009, #48824, #18857 ) ) ;
#41516=( NAMED_UNIT ( * ) SI_UNIT ( $, .STERADIAN. ) SOLID_ANGLE_UNIT ( ) );
#41653=VECTOR ( 'NONE', #36536, 1000.000000000000000 ) ;
#41673=DIRECTION ( 'NONE',  ( 1.000000000000000000, 0.000000000000000000, 0.000000000000000000 ) ) ;
#41795=LINE ( 'NONE', #68852, #23124 ) ;
#42048=DIRECTION ( 'NONE',  ( 0.7071067811865474617, 0.000000000000000000, 0.7071067811865474617 ) ) ;
#42242=DIRECTION ( 'NONE',  ( -0.7071067811865487940, 0.000000000000000000, 0.7071067811865462405 ) ) ;
#42326=ORIENTED_EDGE ( 'NONE', *, *, #37236, .F. ) ;
#42389=VECTOR ( 'NONE', #6705, 1000.000000000000000 ) ;
#42749=VERTEX_POINT ( 'NONE', #46585 ) ;
#42820=DIRECTION ( 'NONE',  ( 0.000000000000000000, 1.000000000000000000, 0.000000000000000000 ) ) ;
#42855=ORIENTED_EDGE ( 'NONE', *, *, #59929, .F. ) ;
#42932=DIRECTION ( 'NONE',  ( -1.000000000000000000, 0.000000000000000000, 0.000000000000000000 ) ) ;
#43140=VECTOR ( 'NONE', #45361, 1000.000000000000000 ) ;
#43169=ADVANCED_FACE ( 'NONE', ( #45651 ), #40706, .F. ) ;
#43279=CYLINDRICAL_SURFACE ( 'NONE', #29154, 4.999999999999997335 ) ;
#43361=EDGE_CURVE ( 'NONE', #51605, #34064, #60046, .T. ) ;
#43485=ORIENTED_EDGE ( 'NONE', *, *, #25032, .F. ) ;
#43628=CARTESIAN_POINT ( 'NONE',  ( -44.99999999999998579, 22.99999999999998579, 4.000000000000000000 ) ) ;
#43771=AXIS2_PLACEMENT_3D ( 'NONE', #13780, #51428, #18718 ) ;
#43992=LINE ( 'NONE', #750, #48264 ) ;
#44038=AXIS2_PLACEMENT_3D ( 'NONE', #4880, #5229, #58681 ) ;
#44325=CARTESIAN_POINT ( 'NONE',  ( -48.00000000000000711, -20.00000000000000355, 4.000000000000000000 ) ) ;
#44422=DIRECTION ( 'NONE',  ( -4.906538933386759377E-15, -0.7071067811865474617, -0.7071067811865474617 ) ) ;
#44451=( GEOMETRIC_REPRESENTATION_CONTEXT ( 3 ) GLOBAL_UNCERTAINTY_ASSIGNED_CONTEXT ( ( #22658 ) ) GLOBAL_UNIT_ASSIGNED_CONTEXT ( ( #50619, #40071, #8770 ) ) REPRESENTATION_CONTEXT ( 'NONE', 'WORKASPACE' ) );
#44501=CARTESIAN_POINT ( 'NONE',  ( 44.99999999999999289, -20.00000000000000355, 4.000000000000000000 ) ) ;
#44558=DIRECTION ( 'NONE',  ( 0.000000000000000000, 0.000000000000000000, 1.000000000000000000 ) ) ;
#44656=EDGE_CURVE ( 'NONE', #2120, #15985, #49782, .T. ) ;
#44924=CARTESIAN_POINT ( 'NONE',  ( -45.00000000000002132, -20.00000000000000355, 0.000000000000000000 ) ) ;
#45361=DIRECTION ( 'NONE',  ( -1.000000000000000000, 0.000000000000000000, 0.000000000000000000 ) ) ;
#45578=EDGE_LOOP ( 'NONE', ( #61664, #67387 ) ) ;
#45651=FACE_OUTER_BOUND ( 'NONE', #15509, .T. ) ;
#45883=EDGE_CURVE ( 'NONE', #7537, #42749, #28433, .T. ) ;
#45903=AXIS2_PLACEMENT_3D ( 'NONE', #54060, #22079, #6943 ) ;
#45946=LINE ( 'NONE', #19560, #33062 ) ;
#46115=ORIENTED_EDGE ( 'NONE', *, *, #58413, .T. ) ;
#46314=EDGE_LOOP ( 'NONE', ( #50436, #23733, #9744, #30193 ) ) ;
#46328=DIRECTION ( 'NONE',  ( 0.000000000000000000, 0.000000000000000000, 1.000000000000000000 ) ) ;
#46447=EDGE_CURVE ( 'NONE', #60851, #34064, #60548, .T. ) ;
#46585=CARTESIAN_POINT ( 'NONE',  ( 49.99999999999998579, 19.99999999999996447, 1.999999999999984457 ) ) ;
#46595=DIRECTION ( 'NONE',  ( 1.000000000000000000, 0.000000000000000000, -0.000000000000000000 ) ) ;
#46669=VECTOR ( 'NONE', #38455, 1000.000000000000000 ) ;
#46720=AXIS2_PLACEMENT_3D ( 'NONE', #7845, #50746, #24022 ) ;
#46902=DIRECTION ( 'NONE',  ( 1.000000000000000000, 0.000000000000000000, 0.000000000000000000 ) ) ;
#46905=ORIENTED_EDGE ( 'NONE', *, *, #8425, .T. ) ;
#47191=AXIS2_PLACEMENT_3D ( 'NONE', #44501, #33262, #6523 ) ;
#47225=AXIS2_PLACEMENT_3D ( 'NONE', #3125, #19282, #24585 ) ;
#47431=ORIENTED_EDGE ( 'NONE', *, *, #12788, .F. ) ;
#47479=DIRECTION ( 'NONE',  ( -0.000000000000000000, -0.000000000000000000, 1.000000000000000000 ) ) ;
#47794=ORIENTED_EDGE ( 'NONE', *, *, #13502, .T. ) ;
#47946=VECTOR ( 'NONE', #15004, 1000.000000000000000 ) ;
#47977=AXIS2_PLACEMENT_3D ( 'NONE', #39135, #12741, #55638 ) ;
#48014=EDGE_CURVE ( 'NONE', #31561, #12851, #25633, .T. ) ;
#48264=VECTOR ( 'NONE', #1098, 1000.000000000000114 ) ;
#48269=VERTEX_POINT ( 'NONE', #4934 ) ;
#48278=CONICAL_SURFACE ( 'NONE', #57309, 2.999999999999981792, 0.7853981633974482790 ) ;
#48370=ORIENTED_EDGE ( 'NONE', *, *, #40498, .F. ) ;
#48504=EDGE_LOOP ( 'NONE', ( #13009, #9800 ) ) ;
#48539=EDGE_CURVE ( 'NONE', #21176, #16065, #64289, .T. ) ;
#48598=ORIENTED_EDGE ( 'NONE', *, *, #13881, .T. ) ;
#48824=ORIENTED_EDGE ( 'NONE', *, *, #27455, .F. ) ;
#49018=DIRECTION ( 'NONE',  ( -0.7071067811865475727, 0.000000000000000000, 0.7071067811865475727 ) ) ;
#49203=EDGE_CURVE ( 'NONE', #10266, #62075, #4223, .T. ) ;
#49484=DIRECTION ( 'NONE',  ( 0.000000000000000000, 0.000000000000000000, -1.000000000000000000 ) ) ;
#49519=ORIENTED_EDGE ( 'NONE', *, *, #986, .T. ) ;
#49630=CARTESIAN_POINT ( 'NONE',  ( -44.29440389294402536, -17.09499999999999886, 4.000000000000000000 ) ) ;
#49686=CARTESIAN_POINT ( 'NONE',  ( -44.29440389294402536, 17.09499999999999886, 4.000000000000000000 ) ) ;
#49782=LINE ( 'NONE', #3009, #5118 ) ;
#49842=ORIENTED_EDGE ( 'NONE', *, *, #25032, .T. ) ;
#50018=CONICAL_SURFACE ( 'NONE', #8459, 2.999999999999981792, 0.7853981633974482790 ) ;
#50180=CARTESIAN_POINT ( 'NONE',  ( 44.99999999999999289, 20.00000000000000355, 2.000000000000015543 ) ) ;
#50261=PLANE ( 'NONE',  #47225 ) ;
#50267=VERTEX_POINT ( 'NONE', #17050 ) ;
#50436=ORIENTED_EDGE ( 'NONE', *, *, #38178, .F. ) ;
#50501=ADVANCED_FACE ( 'NONE', ( #40956 ), #19850, .F. ) ;
#50503=EDGE_LOOP ( 'NONE', ( #39124, #24480, #29421, #29435 ) ) ;
#50530=CARTESIAN_POINT ( 'NONE',  ( 0.000000000000000000, 0.000000000000000000, 0.000000000000000000 ) ) ;
#50619=( LENGTH_UNIT ( ) NAMED_UNIT ( * ) SI_UNIT ( .MILLI., .METRE. ) );
#50666=EDGE_CURVE ( 'NONE', #62075, #10266, #5732, .T. ) ;
#50718=ORIENTED_EDGE ( 'NONE', *, *, #34056, .T. ) ;
#50746=DIRECTION ( 'NONE',  ( -0.000000000000000000, -0.000000000000000000, 1.000000000000000000 ) ) ;
#50769=DIRECTION ( 'NONE',  ( 1.000000000000000000, 0.000000000000000000, 0.000000000000000000 ) ) ;
#50780=CONICAL_SURFACE ( 'NONE', #64282, 4.999999999999997335, 0.7853981633974482790 ) ;
#50939=DIRECTION ( 'NONE',  ( 1.000000000000000000, 0.000000000000000000, 0.000000000000000000 ) ) ;
#51035=FILL_AREA_STYLE ('',( #29570 ) ) ;
#51150=EDGE_CURVE ( 'NONE', #48269, #12851, #471, .T. ) ;
#51323=DIRECTION ( 'NONE',  ( 0.000000000000000000, -0.7071067811865474617, 0.7071067811865474617 ) ) ;
#51428=DIRECTION ( 'NONE',  ( -0.000000000000000000, -0.000000000000000000, 1.000000000000000000 ) ) ;
#51510=LINE ( 'NONE', #19480, #17789 ) ;
#51605=VERTEX_POINT ( 'NONE', #36221 ) ;
#51624=EDGE_CURVE ( 'NONE', #63560, #25708, #57475, .T. ) ;
#51708=ORIENTED_EDGE ( 'NONE', *, *, #31433, .T. ) ;
#51735=ORIENTED_EDGE ( 'NONE', *, *, #44656, .T. ) ;
#51752=PRODUCT_DEFINITION_SHAPE ( 'NONE', 'NONE',  #67192 ) ;
#51936=VECTOR ( 'NONE', #17937, 1000.000000000000000 ) ;
#51946=VECTOR ( 'NONE', #14352, 1000.000000000000114 ) ;
#52340=ORIENTED_EDGE ( 'NONE', *, *, #66483, .F. ) ;
#52413=CARTESIAN_POINT ( 'NONE',  ( 49.99999999999998579, -19.99999999999996447, 1.999999999999984457 ) ) ;
#52454=FACE_OUTER_BOUND ( 'NONE', #41502, .T. ) ;
#52459=DIRECTION ( 'NONE',  ( -1.000000000000000000, 0.000000000000000000, 0.000000000000000000 ) ) ;
#52466=VECTOR ( 'NONE', #42820, 1000.000000000000000 ) ;
#52568=CARTESIAN_POINT ( 'NONE',  ( -39.29440389294403246, -17.09499999999999886, 0.000000000000000000 ) ) ;
#52632=EDGE_CURVE ( 'NONE', #65565, #4244, #63569, .T. ) ;
#52740=SURFACE_SIDE_STYLE ('',( #8475 ) ) ;
#52746=AXIS2_PLACEMENT_3D ( 'NONE', #18580, #61824, #50939 ) ;
#52756=DIRECTION ( 'NONE',  ( 1.000000000000000000, 0.000000000000000000, 0.000000000000000000 ) ) ;
#53319=CARTESIAN_POINT ( 'NONE',  ( 49.99999999999998579, -19.99999999999996447, 1.999999999999984457 ) ) ;
#53424=( LENGTH_UNIT ( ) NAMED_UNIT ( * ) SI_UNIT ( .MILLI., .METRE. ) );
#53453=CARTESIAN_POINT ( 'NONE',  ( 44.99999999999999289, 20.00000000000000355, 2.000000000000015543 ) ) ;
#53470=CIRCLE ( 'NONE', #46720, 4.999999999999997335 ) ;
#53830=APPLICATION_CONTEXT ( 'automotive_design' ) ;
#53921=ORIENTED_EDGE ( 'NONE', *, *, #34056, .F. ) ;
#54060=CARTESIAN_POINT ( 'NONE',  ( -39.29440389294403246, 17.09499999999999886, 4.000000000000000000 ) ) ;
#54281=ORIENTED_EDGE ( 'NONE', *, *, #21271, .F. ) ;
#54413=FACE_OUTER_BOUND ( 'NONE', #20898, .T. ) ;
#54448=LINE ( 'NONE', #33015, #56759 ) ;
#54661=EDGE_LOOP ( 'NONE', ( #63217, #36402, #29271, #4762 ) ) ;
#54855=ORIENTED_EDGE ( 'NONE', *, *, #13214, .T. ) ;
#54925=CARTESIAN_POINT ( 'NONE',  ( -39.29440389294403246, -17.09499999999999886, 4.000000000000000000 ) ) ;
#55043=CIRCLE ( 'NONE', #37074, 4.999999999999997335 ) ;
#55071=ORIENTED_EDGE ( 'NONE', *, *, #986, .F. ) ;
#55138=AXIS2_PLACEMENT_3D ( 'NONE', #12803, #7533, #50769 ) ;
#55186=EDGE_LOOP ( 'NONE', ( #183, #34170 ) ) ;
#55190=ADVANCED_FACE ( 'NONE', ( #16541 ), #32723, .T. ) ;
#55242=CONICAL_SURFACE ( 'NONE', #66524, 4.999999999999997335, 0.7853981633974482790 ) ;
#55354=DIRECTION ( 'NONE',  ( 0.000000000000000000, 0.7071067811865474617, -0.7071067811865474617 ) ) ;
#55410=ORIENTED_EDGE ( 'NONE', *, *, #17127, .T. ) ;
#55498=AXIS2_PLACEMENT_3D ( 'NONE', #65430, #27085, #37642 ) ;
#55638=DIRECTION ( 'NONE',  ( 1.000000000000000000, 0.000000000000000000, 0.000000000000000000 ) ) ;
#55749=DIRECTION ( 'NONE',  ( -1.000000000000000000, 0.000000000000000000, 0.000000000000000000 ) ) ;
#55865=DIRECTION ( 'NONE',  ( 0.7071067811865487940, 0.000000000000000000, 0.7071067811865462405 ) ) ;
#56144=EDGE_CURVE ( 'NONE', #2120, #48269, #61169, .T. ) ;
#56345=ORIENTED_EDGE ( 'NONE', *, *, #36079, .F. ) ;
#56434=ORIENTED_EDGE ( 'NONE', *, *, #8425, .F. ) ;
#56545=CARTESIAN_POINT ( 'NONE',  ( 44.99999999999999289, 20.00000000000000355, 4.000000000000000000 ) ) ;
#56710=CARTESIAN_POINT ( 'NONE',  ( 44.99999999999999289, 22.99999999999998579, 0.000000000000000000 ) ) ;
#56759=VECTOR ( 'NONE', #6275, 1000.000000000000000 ) ;
#57045=CARTESIAN_POINT ( 'NONE',  ( -50.00000000000001421, 19.99999999999996447, 2.000000000000015543 ) ) ;
#57113=DIRECTION ( 'NONE',  ( 1.000000000000000000, 0.000000000000000000, 0.000000000000000000 ) ) ;
#57309=AXIS2_PLACEMENT_3D ( 'NONE', #31687, #25396, #31012 ) ;
#57475=CIRCLE ( 'NONE', #14790, 2.999999999999981792 ) ;
#57482=DIRECTION ( 'NONE',  ( 0.000000000000000000, -0.7071067811865475727, 0.7071067811865475727 ) ) ;
#57858=AXIS2_PLACEMENT_3D ( 'NONE', #67225, #34854, #35540 ) ;
#58117=EDGE_CURVE ( 'NONE', #48269, #39558, #53470, .T. ) ;
#58246=AXIS2_PLACEMENT_3D ( 'NONE', #44924, #23130, #60753 ) ;
#58297=CONICAL_SURFACE ( 'NONE', #26865, 2.999999999999981792, 0.7853981633974482790 ) ;
#58413=EDGE_CURVE ( 'NONE', #12560, #65565, #34389, .T. ) ;
#58515=ORIENTED_EDGE ( 'NONE', *, *, #37236, .T. ) ;
#58681=DIRECTION ( 'NONE',  ( 1.000000000000000000, 0.000000000000000000, 0.000000000000000000 ) ) ;
#58740=STYLED_ITEM ( 'NONE', ( #15809 ), #39790 ) ;
#58809=ADVANCED_FACE ( 'NONE', ( #30780, #40981, #62443 ), #14258, .T. ) ;
#59083=PRODUCT ( 'cutting blade 2', 'cutting blade 2', '', ( #6931 ) ) ;
#59114=LINE ( 'NONE', #11274, #42389 ) ;
#59280=ORIENTED_EDGE ( 'NONE', *, *, #59929, .T. ) ;
#59461=DIRECTION ( 'NONE',  ( -0.000000000000000000, -0.000000000000000000, -1.000000000000000000 ) ) ;
#59591=AXIS2_PLACEMENT_3D ( 'NONE', #50180, #18522, #34365 ) ;
#59640=LINE ( 'NONE', #11454, #4799 ) ;
#59734=DIRECTION ( 'NONE',  ( 1.000000000000000000, 0.000000000000000000, 0.000000000000000000 ) ) ;
#59784=CARTESIAN_POINT ( 'NONE',  ( -45.00000000000000000, 22.99999999999998579, 4.000000000000000000 ) ) ;
#59788=ORIENTED_EDGE ( 'NONE', *, *, #58117, .F. ) ;
#59929=EDGE_CURVE ( 'NONE', #15307, #38832, #41795, .T. ) ;
#59947=ORIENTED_EDGE ( 'NONE', *, *, #13214, .F. ) ;
#60001=VECTOR ( 'NONE', #42048, 1000.000000000000114 ) ;
#60046=CIRCLE ( 'NONE', #66821, 4.999999999999997335 ) ;
#60548=LINE ( 'NONE', #49630, #32238 ) ;
#60603=CYLINDRICAL_SURFACE ( 'NONE', #2643, 4.999999999999997335 ) ;
#60661=LINE ( 'NONE', #18104, #9615 ) ;
#60717=EDGE_LOOP ( 'NONE', ( #49519, #63915, #33077, #35406 ) ) ;
#60726=CARTESIAN_POINT ( 'NONE',  ( 44.99999999999995737, -22.99999999999998579, 0.000000000000000000 ) ) ;
#60753=DIRECTION ( 'NONE',  ( 1.000000000000000000, 0.000000000000000000, 0.000000000000000000 ) ) ;
#60802=FACE_BOUND ( 'NONE', #45578, .T. ) ;
#60851=VERTEX_POINT ( 'NONE', #63607 ) ;
#60906=DIRECTION ( 'NONE',  ( 0.000000000000000000, 0.000000000000000000, 1.000000000000000000 ) ) ;
#60950=CARTESIAN_POINT ( 'NONE',  ( -39.29440389294403246, -17.09499999999999886, 4.000000000000000000 ) ) ;
#61023=FACE_OUTER_BOUND ( 'NONE', #19933, .T. ) ;
#61169=LINE ( 'NONE', #12994, #64542 ) ;
#61339=CARTESIAN_POINT ( 'NONE',  ( -44.99999999999998579, -25.00000000000000000, 2.000000000000015543 ) ) ;
#61511=FACE_OUTER_BOUND ( 'NONE', #35731, .T. ) ;
#61664=ORIENTED_EDGE ( 'NONE', *, *, #36079, .T. ) ;
#61824=DIRECTION ( 'NONE',  ( 0.000000000000000000, 0.000000000000000000, 1.000000000000000000 ) ) ;
#61873=LINE ( 'NONE', #67870, #43140 ) ;
#61882=AXIS2_PLACEMENT_3D ( 'NONE', #39324, #11882, #1336 ) ;
#62019=CARTESIAN_POINT ( 'NONE',  ( -50.00000000000001421, -20.00000000000000355, 1.999999999999984457 ) ) ;
#62051=EDGE_LOOP ( 'NONE', ( #51735, #59947, #54281, #9255 ) ) ;
#62075=VERTEX_POINT ( 'NONE', #2635 ) ;
#62091=CARTESIAN_POINT ( 'NONE',  ( -44.99999999999998579, -22.99999999999998579, 0.000000000000000000 ) ) ;
#62173=CIRCLE ( 'NONE', #30708, 2.999999999999981792 ) ;
#62322=FACE_OUTER_BOUND ( 'NONE', #60717, .T. ) ;
#62363=DIRECTION ( 'NONE',  ( -0.7071067811865474617, 0.000000000000000000, -0.7071067811865474617 ) ) ;
#62443=FACE_BOUND ( 'NONE', #55186, .T. ) ;
#62499=EDGE_CURVE ( 'NONE', #25496, #12560, #68144, .T. ) ;
#62897=CIRCLE ( 'NONE', #13488, 4.999999999999997335 ) ;
#63041=AXIS2_PLACEMENT_3D ( 'NONE', #13538, #57482, #34993 ) ;
#63217=ORIENTED_EDGE ( 'NONE', *, *, #17127, .F. ) ;
#63424=DIRECTION ( 'NONE',  ( -0.000000000000000000, -0.000000000000000000, -1.000000000000000000 ) ) ;
#63560=VERTEX_POINT ( 'NONE', #66691 ) ;
#63569=LINE ( 'NONE', #30184, #51946 ) ;
#63607=CARTESIAN_POINT ( 'NONE',  ( -44.29440389294402536, -17.09499999999999886, 4.000000000000000000 ) ) ;
#63608=ORIENTED_EDGE ( 'NONE', *, *, #52632, .T. ) ;
#63650=DIRECTION ( 'NONE',  ( 1.000000000000000000, 3.700743415417210977E-14, 0.000000000000000000 ) ) ;
#63915=ORIENTED_EDGE ( 'NONE', *, *, #34936, .T. ) ;
#63972=EDGE_LOOP ( 'NONE', ( #38348, #35619, #55071, #12589 ) ) ;
#64039=CARTESIAN_POINT ( 'NONE',  ( 44.99999999999999289, 22.99999999999998579, 4.000000000000000000 ) ) ;
#64096=SHAPE_REPRESENTATION ( 'cutting blade 2', ( #66832 ), #44451 ) ;
#64282=AXIS2_PLACEMENT_3D ( 'NONE', #39737, #1404, #22858 ) ;
#64289=LINE ( 'NONE', #11164, #52466 ) ;
#64337=ORIENTED_EDGE ( 'NONE', *, *, #65380, .T. ) ;
#64375=DIRECTION ( 'NONE',  ( 1.000000000000000000, 0.000000000000000000, -0.000000000000000000 ) ) ;
#64387=CONICAL_SURFACE ( 'NONE', #3745, 4.999999999999997335, 0.7853981633974482790 ) ;
#64399=LINE ( 'NONE', #43628, #12325 ) ;
#64542=VECTOR ( 'NONE', #65053, 1000.000000000000000 ) ;
#64587=ADVANCED_FACE ( 'NONE', ( #23823 ), #58297, .T. ) ;
#64767=CARTESIAN_POINT ( 'NONE',  ( -39.29440389294403246, 17.09499999999999886, 4.000000000000000000 ) ) ;
#65034=CARTESIAN_POINT ( 'NONE',  ( -39.29440389294403246, 17.09499999999999886, 4.000000000000000000 ) ) ;
#65053=DIRECTION ( 'NONE',  ( -1.000000000000000000, 0.000000000000000000, 0.000000000000000000 ) ) ;
#65074=ORIENTED_EDGE ( 'NONE', *, *, #21903, .F. ) ;
#65370=ORIENTED_EDGE ( 'NONE', *, *, #46447, .F. ) ;
#65380=EDGE_CURVE ( 'NONE', #38832, #7537, #10095, .T. ) ;
#65430=CARTESIAN_POINT ( 'NONE',  ( 44.99999999999999289, -22.99999999999998579, 4.000000000000000000 ) ) ;
#65565=VERTEX_POINT ( 'NONE', #38612 ) ;
#65687=ADVANCED_FACE ( 'NONE', ( #52454 ), #48278, .T. ) ;
#65805=ORIENTED_EDGE ( 'NONE', *, *, #56144, .F. ) ;
#65814=CIRCLE ( 'NONE', #1791, 4.999999999999997335 ) ;
#65880=CARTESIAN_POINT ( 'NONE',  ( -48.00000000000000000, 19.99999999999996447, 4.000000000000000000 ) ) ;
#65961=CARTESIAN_POINT ( 'NONE',  ( -48.00000000000000711, -20.00000000000000355, 0.000000000000000000 ) ) ;
#66069=ADVANCED_FACE ( 'NONE', ( #11786 ), #30388, .T. ) ;
#66247=CIRCLE ( 'NONE', #52746, 2.999999999999981792 ) ;
#66257=DIRECTION ( 'NONE',  ( -1.000000000000000000, 0.000000000000000000, 0.000000000000000000 ) ) ;
#66483=EDGE_CURVE ( 'NONE', #12851, #63560, #19766, .T. ) ;
#66524=AXIS2_PLACEMENT_3D ( 'NONE', #39756, #13037, #34500 ) ;
#66691=CARTESIAN_POINT ( 'NONE',  ( 44.99999999999997158, 22.99999999999998579, 0.000000000000000000 ) ) ;
#66749=DIRECTION ( 'NONE',  ( -1.000000000000000000, 0.000000000000000000, 0.000000000000000000 ) ) ;
#66821=AXIS2_PLACEMENT_3D ( 'NONE', #52568, #20217, #41673 ) ;
#66832=AXIS2_PLACEMENT_3D ( 'NONE', #50530, #44558, #8319 ) ;
#67192=PRODUCT_DEFINITION ( 'UNKNOWN', '', #41145, #16253 ) ;
#67202=CARTESIAN_POINT ( 'NONE',  ( 47.99999999999997158, -19.99999999999997868, 0.000000000000000000 ) ) ;
#67225=CARTESIAN_POINT ( 'NONE',  ( 47.99999999999997158, -20.00000000000000355, 4.000000000000000000 ) ) ;
#67261=ORIENTED_EDGE ( 'NONE', *, *, #33113, .T. ) ;
#67313=EDGE_LOOP ( 'NONE', ( #37629, #47794, #21508, #67452 ) ) ;
#67387=ORIENTED_EDGE ( 'NONE', *, *, #43361, .T. ) ;
#67428=ADVANCED_FACE ( 'NONE', ( #38810 ), #60603, .F. ) ;
#67452=ORIENTED_EDGE ( 'NONE', *, *, #23379, .F. ) ;
#67584=EDGE_LOOP ( 'NONE', ( #35135, #32207, #68447, #31432 ) ) ;
#67680=EDGE_CURVE ( 'NONE', #7537, #21176, #14090, .T. ) ;
#67870=CARTESIAN_POINT ( 'NONE',  ( 44.99999999999999289, -22.99999999999998579, 0.000000000000000000 ) ) ;
#67993=ORIENTED_EDGE ( 'NONE', *, *, #32179, .F. ) ;
#68001=CARTESIAN_POINT ( 'NONE',  ( -48.00000000000000000, 19.99999999999996447, 4.000000000000000000 ) ) ;
#68144=LINE ( 'NONE', #26257, #47946 ) ;
#68162=CARTESIAN_POINT ( 'NONE',  ( 44.99999999999997158, 22.99999999999998579, 4.000000000000000000 ) ) ;
#68447=ORIENTED_EDGE ( 'NONE', *, *, #49203, .F. ) ;
#68615=DIRECTION ( 'NONE',  ( -0.000000000000000000, -0.000000000000000000, 1.000000000000000000 ) ) ;
#68770=LINE ( 'NONE', #20585, #60001 ) ;
#68846=VECTOR ( 'NONE', #11124, 1000.000000000000114 ) ;
#68852=CARTESIAN_POINT ( 'NONE',  ( 44.99999999999995737, -22.99999999999998579, 0.000000000000000000 ) ) ;
#68957=PLANE ( 'NONE',  #9426 ) ;
#69065=ORIENTED_EDGE ( 'NONE', *, *, #56144, .T. ) ;
#69275=DIRECTION ( 'NONE',  ( 0.000000000000000000, 0.000000000000000000, 1.000000000000000000 ) ) ;
ENDSEC;
END-ISO-10303-21;
